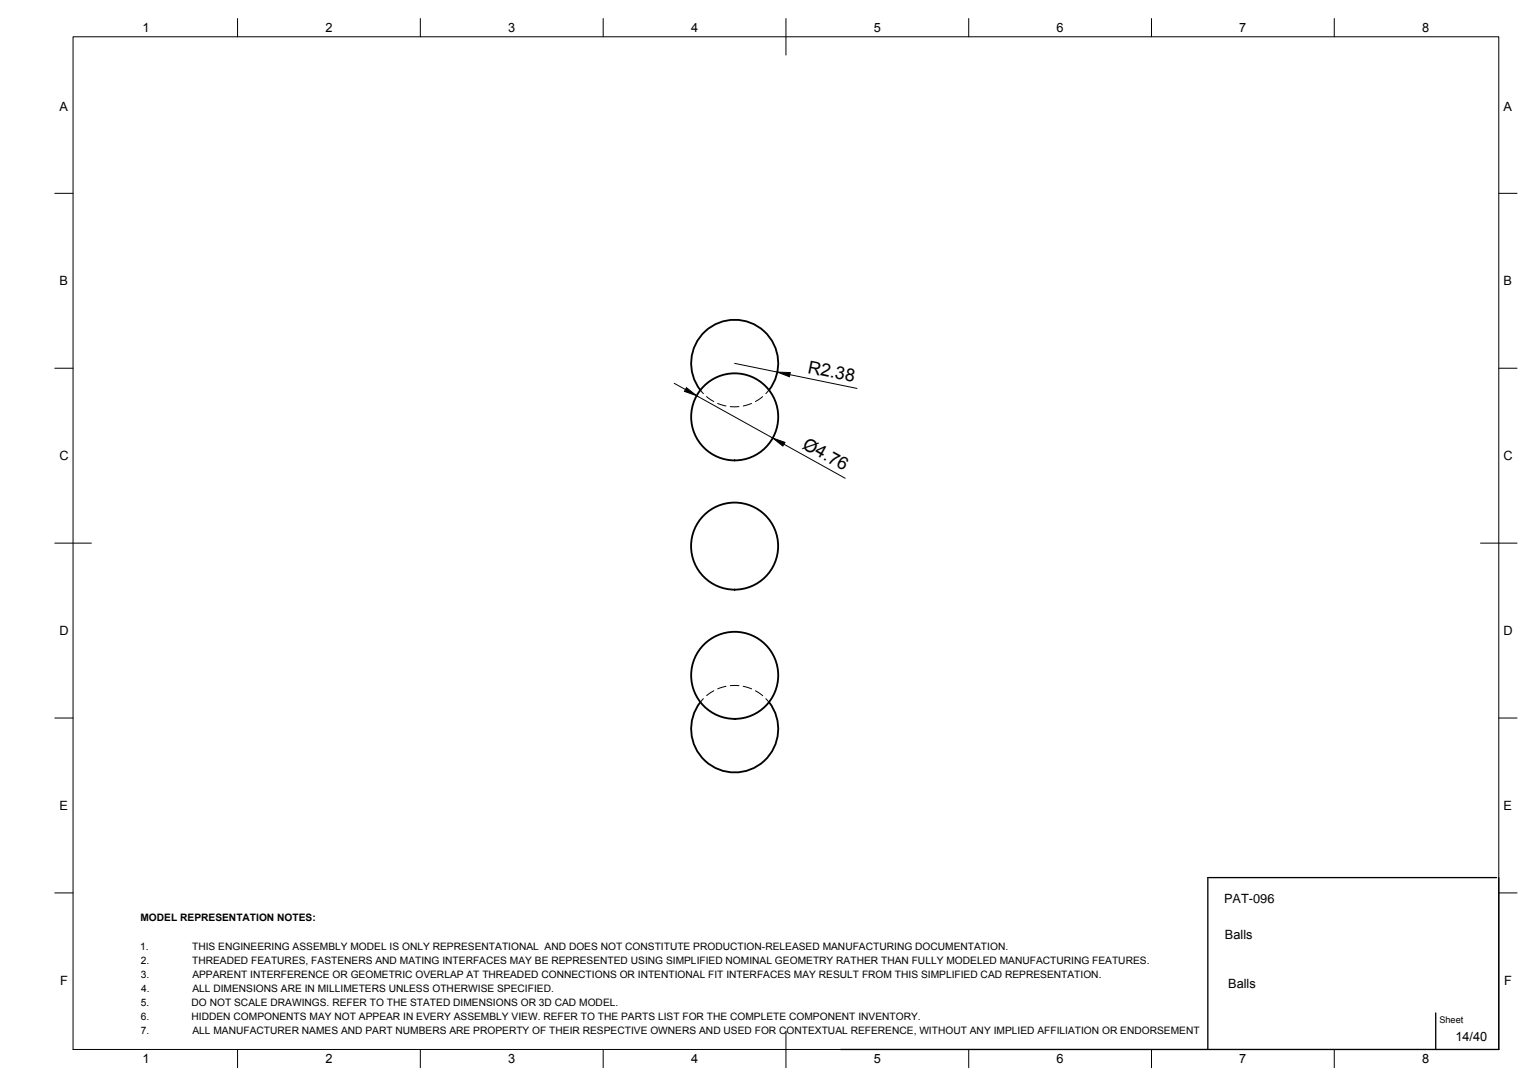
ISO-10303-21;
HEADER;
/* Generated by software containing ST-Developer
 * from STEP Tools, Inc. (www.steptools.com) 
 */

FILE_DESCRIPTION(
/* description */ ('PAT-096'),
/* implementation_level */ '2;1');

FILE_NAME(
/* name */ 'Balls.step',
/* time_stamp */ '2026-10-29T17:03:14-07:00',
/* author */ (''),
/* organization */ (''),
/* preprocessor_version */ 'ST-DEVELOPER v20.2',
/* originating_system */ 'Autodesk Translation Framework v15.17.0.0',
/* authorisation */ '');

FILE_SCHEMA (('AUTOMOTIVE_DESIGN { 1 0 10303 214 3 1 1 }'));
ENDSEC;

DATA;
#10=MECHANICAL_DESIGN_GEOMETRIC_PRESENTATION_REPRESENTATION('',(#404,#405,#406,#407,#408,#409,#410,#411),#10650);
#263=SPHERICAL_SURFACE('',#6125,0.23815);
#264=SPHERICAL_SURFACE('',#6127,0.23815);
#265=SPHERICAL_SURFACE('',#6129,0.23815);
#266=SPHERICAL_SURFACE('',#6131,0.23815);
#267=SPHERICAL_SURFACE('',#6133,0.23815);
#268=SPHERICAL_SURFACE('',#6135,0.23815);
#269=SPHERICAL_SURFACE('',#6137,0.23815);
#270=SPHERICAL_SURFACE('',#6139,0.23815);
#342=SHAPE_REPRESENTATION_RELATIONSHIP('SRR','None',#10803,#373);
#373=ADVANCED_BREP_SHAPE_REPRESENTATION('',(#442,#443,#444,#445,#446,#447,
#448,#449),#10621);
#404=STYLED_ITEM('',(#11064),#442);
#405=STYLED_ITEM('',(#11064),#443);
#406=STYLED_ITEM('',(#11064),#444);
#407=STYLED_ITEM('',(#11064),#445);
#408=STYLED_ITEM('',(#11064),#446);
#409=STYLED_ITEM('',(#11064),#447);
#410=STYLED_ITEM('',(#11064),#448);
#411=STYLED_ITEM('',(#11064),#449);
#442=MANIFOLD_SOLID_BREP('Body1',#5538);
#443=MANIFOLD_SOLID_BREP('Body2',#5539);
#444=MANIFOLD_SOLID_BREP('Body3',#5540);
#445=MANIFOLD_SOLID_BREP('Body4',#5541);
#446=MANIFOLD_SOLID_BREP('Body5',#5542);
#447=MANIFOLD_SOLID_BREP('Body6',#5543);
#448=MANIFOLD_SOLID_BREP('Body7',#5544);
#449=MANIFOLD_SOLID_BREP('Body8',#5545);
#883=FACE_OUTER_BOUND('',#1273,.T.);
#884=FACE_OUTER_BOUND('',#1274,.T.);
#885=FACE_OUTER_BOUND('',#1275,.T.);
#886=FACE_OUTER_BOUND('',#1276,.T.);
#887=FACE_OUTER_BOUND('',#1277,.T.);
#888=FACE_OUTER_BOUND('',#1278,.T.);
#889=FACE_OUTER_BOUND('',#1279,.T.);
#890=FACE_OUTER_BOUND('',#1280,.T.);
#1273=EDGE_LOOP('',(#4107,#4108));
#1274=EDGE_LOOP('',(#4109,#4110));
#1275=EDGE_LOOP('',(#4111,#4112));
#1276=EDGE_LOOP('',(#4113,#4114));
#1277=EDGE_LOOP('',(#4115,#4116));
#1278=EDGE_LOOP('',(#4117,#4118));
#1279=EDGE_LOOP('',(#4119,#4120));
#1280=EDGE_LOOP('',(#4121,#4122));
#2366=CIRCLE('',#6126,0.23815);
#2367=CIRCLE('',#6128,0.23815);
#2368=CIRCLE('',#6130,0.23815);
#2369=CIRCLE('',#6132,0.23815);
#2370=CIRCLE('',#6134,0.23815);
#2371=CIRCLE('',#6136,0.23815);
#2372=CIRCLE('',#6138,0.23815);
#2373=CIRCLE('',#6140,0.23815);
#2707=VERTEX_POINT('',#9009);
#2708=VERTEX_POINT('',#9010);
#2709=VERTEX_POINT('',#9013);
#2710=VERTEX_POINT('',#9014);
#2711=VERTEX_POINT('',#9017);
#2712=VERTEX_POINT('',#9018);
#2713=VERTEX_POINT('',#9021);
#2714=VERTEX_POINT('',#9022);
#2715=VERTEX_POINT('',#9025);
#2716=VERTEX_POINT('',#9026);
#2717=VERTEX_POINT('',#9029);
#2718=VERTEX_POINT('',#9030);
#2719=VERTEX_POINT('',#9033);
#2720=VERTEX_POINT('',#9034);
#2721=VERTEX_POINT('',#9037);
#2722=VERTEX_POINT('',#9038);
#3232=EDGE_CURVE('',#2707,#2708,#2366,.T.);
#3233=EDGE_CURVE('',#2709,#2710,#2367,.T.);
#3234=EDGE_CURVE('',#2711,#2712,#2368,.T.);
#3235=EDGE_CURVE('',#2713,#2714,#2369,.T.);
#3236=EDGE_CURVE('',#2715,#2716,#2370,.T.);
#3237=EDGE_CURVE('',#2717,#2718,#2371,.T.);
#3238=EDGE_CURVE('',#2719,#2720,#2372,.T.);
#3239=EDGE_CURVE('',#2721,#2722,#2373,.T.);
#4107=ORIENTED_EDGE('',*,*,#3232,.T.);
#4108=ORIENTED_EDGE('',*,*,#3232,.F.);
#4109=ORIENTED_EDGE('',*,*,#3233,.T.);
#4110=ORIENTED_EDGE('',*,*,#3233,.F.);
#4111=ORIENTED_EDGE('',*,*,#3234,.T.);
#4112=ORIENTED_EDGE('',*,*,#3234,.F.);
#4113=ORIENTED_EDGE('',*,*,#3235,.T.);
#4114=ORIENTED_EDGE('',*,*,#3235,.F.);
#4115=ORIENTED_EDGE('',*,*,#3236,.T.);
#4116=ORIENTED_EDGE('',*,*,#3236,.F.);
#4117=ORIENTED_EDGE('',*,*,#3237,.T.);
#4118=ORIENTED_EDGE('',*,*,#3237,.F.);
#4119=ORIENTED_EDGE('',*,*,#3238,.T.);
#4120=ORIENTED_EDGE('',*,*,#3238,.F.);
#4121=ORIENTED_EDGE('',*,*,#3239,.T.);
#4122=ORIENTED_EDGE('',*,*,#3239,.F.);
#5288=ADVANCED_FACE('',(#883),#263,.T.);
#5289=ADVANCED_FACE('',(#884),#264,.T.);
#5290=ADVANCED_FACE('',(#885),#265,.T.);
#5291=ADVANCED_FACE('',(#886),#266,.T.);
#5292=ADVANCED_FACE('',(#887),#267,.T.);
#5293=ADVANCED_FACE('',(#888),#268,.T.);
#5294=ADVANCED_FACE('',(#889),#269,.T.);
#5295=ADVANCED_FACE('',(#890),#270,.T.);
#5538=CLOSED_SHELL('',(#5288));
#5539=CLOSED_SHELL('',(#5289));
#5540=CLOSED_SHELL('',(#5290));
#5541=CLOSED_SHELL('',(#5291));
#5542=CLOSED_SHELL('',(#5292));
#5543=CLOSED_SHELL('',(#5293));
#5544=CLOSED_SHELL('',(#5294));
#5545=CLOSED_SHELL('',(#5295));
#6124=AXIS2_PLACEMENT_3D('',#9007,#7174,#7175);
#6125=AXIS2_PLACEMENT_3D('',#9008,#7176,#7177);
#6126=AXIS2_PLACEMENT_3D('',#9011,#7178,#7179);
#6127=AXIS2_PLACEMENT_3D('',#9012,#7180,#7181);
#6128=AXIS2_PLACEMENT_3D('',#9015,#7182,#7183);
#6129=AXIS2_PLACEMENT_3D('',#9016,#7184,#7185);
#6130=AXIS2_PLACEMENT_3D('',#9019,#7186,#7187);
#6131=AXIS2_PLACEMENT_3D('',#9020,#7188,#7189);
#6132=AXIS2_PLACEMENT_3D('',#9023,#7190,#7191);
#6133=AXIS2_PLACEMENT_3D('',#9024,#7192,#7193);
#6134=AXIS2_PLACEMENT_3D('',#9027,#7194,#7195);
#6135=AXIS2_PLACEMENT_3D('',#9028,#7196,#7197);
#6136=AXIS2_PLACEMENT_3D('',#9031,#7198,#7199);
#6137=AXIS2_PLACEMENT_3D('',#9032,#7200,#7201);
#6138=AXIS2_PLACEMENT_3D('',#9035,#7202,#7203);
#6139=AXIS2_PLACEMENT_3D('',#9036,#7204,#7205);
#6140=AXIS2_PLACEMENT_3D('',#9039,#7206,#7207);
#7174=DIRECTION('axis',(0.,0.,1.));
#7175=DIRECTION('refdir',(1.,0.,0.));
#7176=DIRECTION('center_axis',(0.,0.,1.));
#7177=DIRECTION('ref_axis',(1.,0.,0.));
#7178=DIRECTION('center_axis',(1.22464679914735E-16,-1.,0.));
#7179=DIRECTION('ref_axis',(-1.,-1.22464679914735E-16,0.));
#7180=DIRECTION('center_axis',(0.707106781186548,0.,0.707106781186548));
#7181=DIRECTION('ref_axis',(0.707106781186548,0.,-0.707106781186548));
#7182=DIRECTION('center_axis',(8.65956056235494E-17,-1.,-8.65956056235493E-17));
#7183=DIRECTION('ref_axis',(-0.707106781186547,-1.22464679914735E-16,0.707106781186547));
#7184=DIRECTION('center_axis',(1.,0.,0.));
#7185=DIRECTION('ref_axis',(6.12323399573676E-17,0.,-1.));
#7186=DIRECTION('center_axis',(7.49879891330929E-33,-1.,-1.22464679914735E-16));
#7187=DIRECTION('ref_axis',(-6.12323399573676E-17,-1.22464679914735E-16,
1.));
#7188=DIRECTION('center_axis',(0.707106781186548,0.,-0.707106781186548));
#7189=DIRECTION('ref_axis',(-0.707106781186548,0.,-0.707106781186548));
#7190=DIRECTION('center_axis',(-8.65956056235493E-17,-1.,-8.65956056235494E-17));
#7191=DIRECTION('ref_axis',(0.707106781186547,-1.22464679914735E-16,0.707106781186547));
#7192=DIRECTION('center_axis',(0.,0.,-1.));
#7193=DIRECTION('ref_axis',(-1.,0.,-1.22464679914735E-16));
#7194=DIRECTION('center_axis',(-1.22464679914735E-16,-1.,-1.49975978266186E-32));
#7195=DIRECTION('ref_axis',(1.,-1.22464679914735E-16,1.22464679914735E-16));
#7196=DIRECTION('center_axis',(-0.707106781186547,0.,-0.707106781186548));
#7197=DIRECTION('ref_axis',(-0.707106781186548,0.,0.707106781186547));
#7198=DIRECTION('center_axis',(-8.65956056235493E-17,-1.,8.65956056235493E-17));
#7199=DIRECTION('ref_axis',(0.707106781186548,-1.22464679914735E-16,-0.707106781186547));
#7200=DIRECTION('center_axis',(-1.,0.,0.));
#7201=DIRECTION('ref_axis',(-1.83697019872103E-16,0.,1.));
#7202=DIRECTION('center_axis',(-2.24963967399279E-32,-1.,1.22464679914735E-16));
#7203=DIRECTION('ref_axis',(1.83697019872103E-16,-1.22464679914735E-16,
-1.));
#7204=DIRECTION('center_axis',(-0.707106781186548,0.,0.707106781186548));
#7205=DIRECTION('ref_axis',(0.707106781186547,0.,0.707106781186548));
#7206=DIRECTION('center_axis',(8.65956056235493E-17,-1.,8.65956056235493E-17));
#7207=DIRECTION('ref_axis',(-0.707106781186547,-1.22464679914735E-16,-0.707106781186548));
#9007=CARTESIAN_POINT('',(0.,0.,0.));
#9008=CARTESIAN_POINT('Origin',(1.,0.,0.));
#9009=CARTESIAN_POINT('',(1.,-1.78583896120461E-33,0.23815));
#9010=CARTESIAN_POINT('',(1.,-1.78583896120461E-33,-0.23815));
#9011=CARTESIAN_POINT('Origin',(1.,0.,0.));
#9012=CARTESIAN_POINT('Origin',(0.707106781186548,0.,-0.707106781186547));
#9013=CARTESIAN_POINT('',(0.875504261126124,-1.78583896120461E-33,-0.538709301246971));
#9014=CARTESIAN_POINT('',(0.538709301246971,-1.78583896120461E-33,-0.875504261126124));
#9015=CARTESIAN_POINT('Origin',(0.707106781186548,0.,-0.707106781186547));
#9016=CARTESIAN_POINT('Origin',(6.12323399573677E-17,0.,-1.));
#9017=CARTESIAN_POINT('',(0.23815,-1.78583896120461E-33,-1.));
#9018=CARTESIAN_POINT('',(-0.23815,-1.78583896120461E-33,-1.));
#9019=CARTESIAN_POINT('Origin',(6.12323399573677E-17,0.,-1.));
#9020=CARTESIAN_POINT('Origin',(-0.707106781186547,0.,-0.707106781186548));
#9021=CARTESIAN_POINT('',(-0.538709301246971,-1.78583896120461E-33,-0.875504261126124));
#9022=CARTESIAN_POINT('',(-0.875504261126124,-1.78583896120461E-33,-0.538709301246971));
#9023=CARTESIAN_POINT('Origin',(-0.707106781186547,0.,-0.707106781186548));
#9024=CARTESIAN_POINT('Origin',(-1.,0.,-1.22464679914735E-16));
#9025=CARTESIAN_POINT('',(-1.,-1.78583896120461E-33,-0.23815));
#9026=CARTESIAN_POINT('',(-1.,-1.78583896120461E-33,0.23815));
#9027=CARTESIAN_POINT('Origin',(-1.,0.,-1.22464679914735E-16));
#9028=CARTESIAN_POINT('Origin',(-0.707106781186548,0.,0.707106781186547));
#9029=CARTESIAN_POINT('',(-0.875504261126124,-7.94881478324376E-33,0.538709301246971));
#9030=CARTESIAN_POINT('',(-0.538709301246971,4.37713686083455E-33,0.875504261126124));
#9031=CARTESIAN_POINT('Origin',(-0.707106781186548,0.,0.707106781186547));
#9032=CARTESIAN_POINT('Origin',(-1.83697019872103E-16,0.,1.));
#9033=CARTESIAN_POINT('',(-0.23815,-1.78583896120461E-33,1.));
#9034=CARTESIAN_POINT('',(0.23815,-1.78583896120461E-33,1.));
#9035=CARTESIAN_POINT('Origin',(-1.83697019872103E-16,0.,1.));
#9036=CARTESIAN_POINT('Origin',(0.707106781186547,0.,0.707106781186548));
#9037=CARTESIAN_POINT('',(0.538709301246971,-4.86732687222419E-33,0.875504261126124));
#9038=CARTESIAN_POINT('',(0.875504261126124,1.29564894981497E-33,0.538709301246971));
#9039=CARTESIAN_POINT('Origin',(0.707106781186547,0.,0.707106781186548));
#10582=UNCERTAINTY_MEASURE_WITH_UNIT(LENGTH_MEASURE(0.001),#10651,
'DISTANCE_ACCURACY_VALUE',
'Maximum model space distance between geometric entities at asserted c
onnectivities');
#10611=UNCERTAINTY_MEASURE_WITH_UNIT(LENGTH_MEASURE(0.001),#10651,
'DISTANCE_ACCURACY_VALUE',
'Maximum model space distance between geometric entities at asserted c
onnectivities');
#10621=(
GEOMETRIC_REPRESENTATION_CONTEXT(3)
GLOBAL_UNCERTAINTY_ASSIGNED_CONTEXT((#10582))
GLOBAL_UNIT_ASSIGNED_CONTEXT((#10651,#10653,#10654))
REPRESENTATION_CONTEXT('','3D')
);
#10650=(
GEOMETRIC_REPRESENTATION_CONTEXT(3)
GLOBAL_UNCERTAINTY_ASSIGNED_CONTEXT((#10611))
GLOBAL_UNIT_ASSIGNED_CONTEXT((#10651,#10653,#10654))
REPRESENTATION_CONTEXT('','3D')
);
#10651=(
LENGTH_UNIT()
NAMED_UNIT(*)
SI_UNIT(.CENTI.,.METRE.)
);
#10653=(
NAMED_UNIT(*)
PLANE_ANGLE_UNIT()
SI_UNIT($,.RADIAN.)
);
#10654=(
NAMED_UNIT(*)
SI_UNIT($,.STERADIAN.)
SOLID_ANGLE_UNIT()
);
#10664=SHAPE_DEFINITION_REPRESENTATION(#10702,#10803);
#10702=PRODUCT_DEFINITION_SHAPE('',$,#10842);
#10803=SHAPE_REPRESENTATION('',(#6124),#10621);
#10832=PRODUCT_DEFINITION_CONTEXT('part definition',#10948,'design');
#10842=PRODUCT_DEFINITION('Balls','Balls',#10880,#10832);
#10880=PRODUCT_DEFINITION_FORMATION('',$,#10959);
#10948=APPLICATION_CONTEXT(
'Core Data for Automotive Mechanical Design Process');
#10949=PRODUCT_CONTEXT('part definition',#10948,'mechanical');
#10959=PRODUCT('Balls','Balls','Balls',(#10949));
#11058=COLOUR_RGB('Grey',0.48,0.52,0.57);
#11059=FILL_AREA_STYLE_COLOUR('',#11058);
#11060=FILL_AREA_STYLE('',(#11059));
#11061=SURFACE_STYLE_FILL_AREA(#11060);
#11062=SURFACE_SIDE_STYLE('',(#11061));
#11063=SURFACE_STYLE_USAGE(.BOTH.,#11062);
#11064=PRESENTATION_STYLE_ASSIGNMENT((#11063));
ENDSEC;
END-ISO-10303-21;
